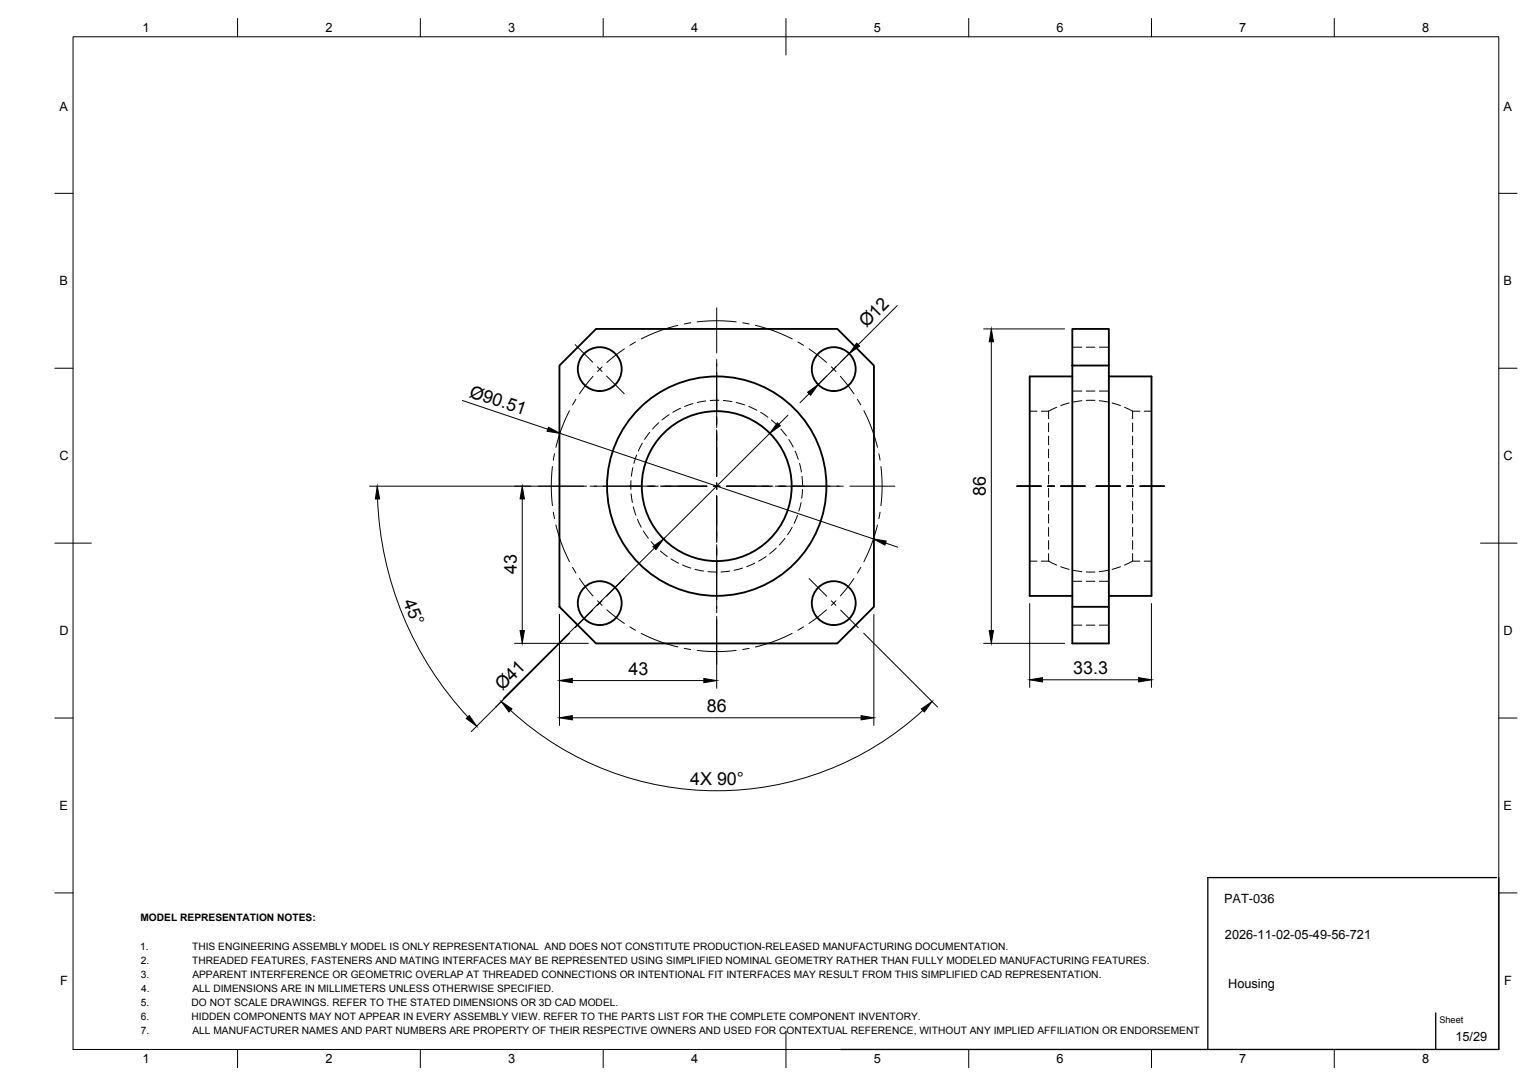
ISO-10303-21;
HEADER;
/* Generated by software containing ST-Developer
 * from STEP Tools, Inc. (www.steptools.com) 
 */

FILE_DESCRIPTION(
/* description */ ('Flange-mounted spindle'),
/* implementation_level */ '2;1');

FILE_NAME(
/* name */ 'Housing.step',
/* time_stamp */ '2026-10-27T10:49:51-07:00',
/* author */ (''),
/* organization */ (''),
/* preprocessor_version */ 'ST-DEVELOPER v20.2',
/* originating_system */ 'Autodesk Translation Framework v15.17.0.0',
/* authorisation */ '');

FILE_SCHEMA (('AUTOMOTIVE_DESIGN { 1 0 10303 214 3 1 1 }'));
ENDSEC;

DATA;
#10=MECHANICAL_DESIGN_GEOMETRIC_PRESENTATION_REPRESENTATION('',(#347),#11764);
#261=SPHERICAL_SURFACE('',#6586,2.35);
#293=SHAPE_REPRESENTATION_RELATIONSHIP('SRR','None',#11890,#320);
#320=ADVANCED_BREP_SHAPE_REPRESENTATION('',(#374),#11745);
#347=STYLED_ITEM('',(#12078),#374);
#374=MANIFOLD_SOLID_BREP('Body1',#6140);
#418=FACE_BOUND('',#1116,.T.);
#419=FACE_BOUND('',#1117,.T.);
#420=FACE_BOUND('',#1121,.T.);
#421=FACE_BOUND('',#1123,.T.);
#422=FACE_BOUND('',#1137,.T.);
#423=FACE_BOUND('',#1138,.T.);
#424=FACE_BOUND('',#1139,.T.);
#425=FACE_BOUND('',#1140,.T.);
#426=FACE_BOUND('',#1141,.T.);
#427=FACE_BOUND('',#1143,.T.);
#428=FACE_BOUND('',#1144,.T.);
#429=FACE_BOUND('',#1145,.T.);
#430=FACE_BOUND('',#1146,.T.);
#431=FACE_BOUND('',#1147,.T.);
#551=PLANE('',#6594);
#552=PLANE('',#6595);
#553=PLANE('',#6608);
#554=PLANE('',#6609);
#555=PLANE('',#6610);
#556=PLANE('',#6611);
#557=PLANE('',#6612);
#558=PLANE('',#6613);
#559=PLANE('',#6614);
#560=PLANE('',#6615);
#561=PLANE('',#6616);
#562=PLANE('',#6617);
#741=FACE_OUTER_BOUND('',#1113,.T.);
#742=FACE_OUTER_BOUND('',#1114,.T.);
#743=FACE_OUTER_BOUND('',#1115,.T.);
#744=FACE_OUTER_BOUND('',#1118,.T.);
#745=FACE_OUTER_BOUND('',#1119,.T.);
#746=FACE_OUTER_BOUND('',#1120,.T.);
#747=FACE_OUTER_BOUND('',#1122,.T.);
#748=FACE_OUTER_BOUND('',#1124,.T.);
#749=FACE_OUTER_BOUND('',#1125,.T.);
#750=FACE_OUTER_BOUND('',#1126,.T.);
#751=FACE_OUTER_BOUND('',#1127,.T.);
#752=FACE_OUTER_BOUND('',#1128,.T.);
#753=FACE_OUTER_BOUND('',#1129,.T.);
#754=FACE_OUTER_BOUND('',#1130,.T.);
#755=FACE_OUTER_BOUND('',#1131,.T.);
#756=FACE_OUTER_BOUND('',#1132,.T.);
#757=FACE_OUTER_BOUND('',#1133,.T.);
#758=FACE_OUTER_BOUND('',#1134,.T.);
#759=FACE_OUTER_BOUND('',#1135,.T.);
#760=FACE_OUTER_BOUND('',#1136,.T.);
#761=FACE_OUTER_BOUND('',#1142,.T.);
#1113=EDGE_LOOP('',(#4275,#4276,#4277,#4278));
#1114=EDGE_LOOP('',(#4279,#4280,#4281,#4282));
#1115=EDGE_LOOP('',(#4283,#4284));
#1116=EDGE_LOOP('',(#4285));
#1117=EDGE_LOOP('',(#4286));
#1118=EDGE_LOOP('',(#4287,#4288,#4289,#4290));
#1119=EDGE_LOOP('',(#4291,#4292,#4293,#4294));
#1120=EDGE_LOOP('',(#4295));
#1121=EDGE_LOOP('',(#4296));
#1122=EDGE_LOOP('',(#4297));
#1123=EDGE_LOOP('',(#4298));
#1124=EDGE_LOOP('',(#4299,#4300,#4301,#4302));
#1125=EDGE_LOOP('',(#4303,#4304,#4305,#4306));
#1126=EDGE_LOOP('',(#4307,#4308,#4309,#4310));
#1127=EDGE_LOOP('',(#4311,#4312,#4313,#4314));
#1128=EDGE_LOOP('',(#4315,#4316,#4317,#4318));
#1129=EDGE_LOOP('',(#4319,#4320,#4321,#4322));
#1130=EDGE_LOOP('',(#4323,#4324,#4325,#4326));
#1131=EDGE_LOOP('',(#4327,#4328,#4329,#4330));
#1132=EDGE_LOOP('',(#4331,#4332,#4333,#4334));
#1133=EDGE_LOOP('',(#4335,#4336,#4337,#4338));
#1134=EDGE_LOOP('',(#4339,#4340,#4341,#4342));
#1135=EDGE_LOOP('',(#4343,#4344,#4345,#4346));
#1136=EDGE_LOOP('',(#4347,#4348,#4349,#4350,#4351,#4352,#4353,#4354));
#1137=EDGE_LOOP('',(#4355));
#1138=EDGE_LOOP('',(#4356));
#1139=EDGE_LOOP('',(#4357));
#1140=EDGE_LOOP('',(#4358));
#1141=EDGE_LOOP('',(#4359));
#1142=EDGE_LOOP('',(#4360,#4361,#4362,#4363,#4364,#4365,#4366,#4367));
#1143=EDGE_LOOP('',(#4368));
#1144=EDGE_LOOP('',(#4369));
#1145=EDGE_LOOP('',(#4370));
#1146=EDGE_LOOP('',(#4371));
#1147=EDGE_LOOP('',(#4372));
#1573=LINE('',#9436,#1995);
#1574=LINE('',#9442,#1996);
#1575=LINE('',#9452,#1997);
#1576=LINE('',#9458,#1998);
#1577=LINE('',#9466,#1999);
#1578=LINE('',#9472,#2000);
#1579=LINE('',#9478,#2001);
#1580=LINE('',#9484,#2002);
#1581=LINE('',#9489,#2003);
#1582=LINE('',#9491,#2004);
#1583=LINE('',#9493,#2005);
#1584=LINE('',#9494,#2006);
#1585=LINE('',#9497,#2007);
#1586=LINE('',#9499,#2008);
#1587=LINE('',#9500,#2009);
#1588=LINE('',#9503,#2010);
#1589=LINE('',#9505,#2011);
#1590=LINE('',#9506,#2012);
#1591=LINE('',#9509,#2013);
#1592=LINE('',#9511,#2014);
#1593=LINE('',#9512,#2015);
#1594=LINE('',#9515,#2016);
#1595=LINE('',#9517,#2017);
#1596=LINE('',#9518,#2018);
#1597=LINE('',#9521,#2019);
#1598=LINE('',#9523,#2020);
#1599=LINE('',#9524,#2021);
#1600=LINE('',#9527,#2022);
#1601=LINE('',#9529,#2023);
#1602=LINE('',#9530,#2024);
#1603=LINE('',#9532,#2025);
#1604=LINE('',#9533,#2026);
#1995=VECTOR('',#7548,2.05);
#1996=VECTOR('',#7555,2.05);
#1997=VECTOR('',#7566,3.);
#1998=VECTOR('',#7573,3.);
#1999=VECTOR('',#7584,0.6);
#2000=VECTOR('',#7591,0.6);
#2001=VECTOR('',#7598,0.6);
#2002=VECTOR('',#7605,0.6);
#2003=VECTOR('',#7610,1.);
#2004=VECTOR('',#7611,1.);
#2005=VECTOR('',#7612,1.);
#2006=VECTOR('',#7613,1.);
#2007=VECTOR('',#7616,1.);
#2008=VECTOR('',#7617,1.);
#2009=VECTOR('',#7618,1.);
#2010=VECTOR('',#7621,1.);
#2011=VECTOR('',#7622,1.);
#2012=VECTOR('',#7623,1.);
#2013=VECTOR('',#7626,1.);
#2014=VECTOR('',#7627,1.);
#2015=VECTOR('',#7628,1.);
#2016=VECTOR('',#7631,1.);
#2017=VECTOR('',#7632,1.);
#2018=VECTOR('',#7633,1.);
#2019=VECTOR('',#7636,1.);
#2020=VECTOR('',#7637,1.);
#2021=VECTOR('',#7638,1.);
#2022=VECTOR('',#7641,1.);
#2023=VECTOR('',#7642,1.);
#2024=VECTOR('',#7643,1.);
#2025=VECTOR('',#7646,1.);
#2026=VECTOR('',#7647,1.);
#2364=CIRCLE('',#6581,2.05);
#2365=CIRCLE('',#6582,2.05);
#2366=CIRCLE('',#6584,2.05);
#2367=CIRCLE('',#6585,2.05);
#2368=CIRCLE('',#6587,2.35);
#2369=CIRCLE('',#6589,3.);
#2370=CIRCLE('',#6590,3.);
#2371=CIRCLE('',#6592,3.);
#2372=CIRCLE('',#6593,3.);
#2373=CIRCLE('',#6597,0.6);
#2374=CIRCLE('',#6598,0.6);
#2375=CIRCLE('',#6600,0.6);
#2376=CIRCLE('',#6601,0.6);
#2377=CIRCLE('',#6603,0.6);
#2378=CIRCLE('',#6604,0.6);
#2379=CIRCLE('',#6606,0.6);
#2380=CIRCLE('',#6607,0.6);
#2738=VERTEX_POINT('',#9433);
#2739=VERTEX_POINT('',#9435);
#2740=VERTEX_POINT('',#9439);
#2741=VERTEX_POINT('',#9441);
#2742=VERTEX_POINT('',#9445);
#2743=VERTEX_POINT('',#9446);
#2744=VERTEX_POINT('',#9449);
#2745=VERTEX_POINT('',#9451);
#2746=VERTEX_POINT('',#9455);
#2747=VERTEX_POINT('',#9457);
#2748=VERTEX_POINT('',#9463);
#2749=VERTEX_POINT('',#9465);
#2750=VERTEX_POINT('',#9469);
#2751=VERTEX_POINT('',#9471);
#2752=VERTEX_POINT('',#9475);
#2753=VERTEX_POINT('',#9477);
#2754=VERTEX_POINT('',#9481);
#2755=VERTEX_POINT('',#9483);
#2756=VERTEX_POINT('',#9487);
#2757=VERTEX_POINT('',#9488);
#2758=VERTEX_POINT('',#9490);
#2759=VERTEX_POINT('',#9492);
#2760=VERTEX_POINT('',#9496);
#2761=VERTEX_POINT('',#9498);
#2762=VERTEX_POINT('',#9502);
#2763=VERTEX_POINT('',#9504);
#2764=VERTEX_POINT('',#9508);
#2765=VERTEX_POINT('',#9510);
#2766=VERTEX_POINT('',#9514);
#2767=VERTEX_POINT('',#9516);
#2768=VERTEX_POINT('',#9520);
#2769=VERTEX_POINT('',#9522);
#2770=VERTEX_POINT('',#9526);
#2771=VERTEX_POINT('',#9528);
#3330=EDGE_CURVE('',#2738,#2738,#2364,.T.);
#3331=EDGE_CURVE('',#2738,#2739,#1573,.T.);
#3332=EDGE_CURVE('',#2739,#2739,#2365,.T.);
#3333=EDGE_CURVE('',#2740,#2740,#2366,.T.);
#3334=EDGE_CURVE('',#2740,#2741,#1574,.T.);
#3335=EDGE_CURVE('',#2741,#2741,#2367,.T.);
#3336=EDGE_CURVE('',#2742,#2743,#2368,.T.);
#3337=EDGE_CURVE('',#2744,#2744,#2369,.T.);
#3338=EDGE_CURVE('',#2744,#2745,#1575,.T.);
#3339=EDGE_CURVE('',#2745,#2745,#2370,.T.);
#3340=EDGE_CURVE('',#2746,#2746,#2371,.T.);
#3341=EDGE_CURVE('',#2746,#2747,#1576,.T.);
#3342=EDGE_CURVE('',#2747,#2747,#2372,.T.);
#3343=EDGE_CURVE('',#2748,#2748,#2373,.T.);
#3344=EDGE_CURVE('',#2748,#2749,#1577,.T.);
#3345=EDGE_CURVE('',#2749,#2749,#2374,.T.);
#3346=EDGE_CURVE('',#2750,#2750,#2375,.T.);
#3347=EDGE_CURVE('',#2750,#2751,#1578,.T.);
#3348=EDGE_CURVE('',#2751,#2751,#2376,.T.);
#3349=EDGE_CURVE('',#2752,#2752,#2377,.T.);
#3350=EDGE_CURVE('',#2752,#2753,#1579,.T.);
#3351=EDGE_CURVE('',#2753,#2753,#2378,.T.);
#3352=EDGE_CURVE('',#2754,#2754,#2379,.T.);
#3353=EDGE_CURVE('',#2754,#2755,#1580,.T.);
#3354=EDGE_CURVE('',#2755,#2755,#2380,.T.);
#3355=EDGE_CURVE('',#2756,#2757,#1581,.T.);
#3356=EDGE_CURVE('',#2757,#2758,#1582,.T.);
#3357=EDGE_CURVE('',#2759,#2758,#1583,.T.);
#3358=EDGE_CURVE('',#2756,#2759,#1584,.T.);
#3359=EDGE_CURVE('',#2760,#2756,#1585,.T.);
#3360=EDGE_CURVE('',#2761,#2759,#1586,.T.);
#3361=EDGE_CURVE('',#2760,#2761,#1587,.T.);
#3362=EDGE_CURVE('',#2762,#2760,#1588,.T.);
#3363=EDGE_CURVE('',#2763,#2761,#1589,.T.);
#3364=EDGE_CURVE('',#2762,#2763,#1590,.T.);
#3365=EDGE_CURVE('',#2764,#2762,#1591,.T.);
#3366=EDGE_CURVE('',#2765,#2763,#1592,.T.);
#3367=EDGE_CURVE('',#2764,#2765,#1593,.T.);
#3368=EDGE_CURVE('',#2766,#2764,#1594,.T.);
#3369=EDGE_CURVE('',#2767,#2765,#1595,.T.);
#3370=EDGE_CURVE('',#2766,#2767,#1596,.T.);
#3371=EDGE_CURVE('',#2768,#2766,#1597,.T.);
#3372=EDGE_CURVE('',#2769,#2767,#1598,.T.);
#3373=EDGE_CURVE('',#2768,#2769,#1599,.T.);
#3374=EDGE_CURVE('',#2770,#2768,#1600,.T.);
#3375=EDGE_CURVE('',#2771,#2769,#1601,.T.);
#3376=EDGE_CURVE('',#2770,#2771,#1602,.T.);
#3377=EDGE_CURVE('',#2757,#2770,#1603,.T.);
#3378=EDGE_CURVE('',#2758,#2771,#1604,.T.);
#4275=ORIENTED_EDGE('',*,*,#3330,.F.);
#4276=ORIENTED_EDGE('',*,*,#3331,.T.);
#4277=ORIENTED_EDGE('',*,*,#3332,.F.);
#4278=ORIENTED_EDGE('',*,*,#3331,.F.);
#4279=ORIENTED_EDGE('',*,*,#3333,.F.);
#4280=ORIENTED_EDGE('',*,*,#3334,.T.);
#4281=ORIENTED_EDGE('',*,*,#3335,.F.);
#4282=ORIENTED_EDGE('',*,*,#3334,.F.);
#4283=ORIENTED_EDGE('',*,*,#3336,.T.);
#4284=ORIENTED_EDGE('',*,*,#3336,.F.);
#4285=ORIENTED_EDGE('',*,*,#3333,.T.);
#4286=ORIENTED_EDGE('',*,*,#3332,.T.);
#4287=ORIENTED_EDGE('',*,*,#3337,.F.);
#4288=ORIENTED_EDGE('',*,*,#3338,.T.);
#4289=ORIENTED_EDGE('',*,*,#3339,.F.);
#4290=ORIENTED_EDGE('',*,*,#3338,.F.);
#4291=ORIENTED_EDGE('',*,*,#3340,.F.);
#4292=ORIENTED_EDGE('',*,*,#3341,.T.);
#4293=ORIENTED_EDGE('',*,*,#3342,.F.);
#4294=ORIENTED_EDGE('',*,*,#3341,.F.);
#4295=ORIENTED_EDGE('',*,*,#3339,.T.);
#4296=ORIENTED_EDGE('',*,*,#3330,.T.);
#4297=ORIENTED_EDGE('',*,*,#3340,.T.);
#4298=ORIENTED_EDGE('',*,*,#3335,.T.);
#4299=ORIENTED_EDGE('',*,*,#3343,.F.);
#4300=ORIENTED_EDGE('',*,*,#3344,.T.);
#4301=ORIENTED_EDGE('',*,*,#3345,.F.);
#4302=ORIENTED_EDGE('',*,*,#3344,.F.);
#4303=ORIENTED_EDGE('',*,*,#3346,.F.);
#4304=ORIENTED_EDGE('',*,*,#3347,.T.);
#4305=ORIENTED_EDGE('',*,*,#3348,.F.);
#4306=ORIENTED_EDGE('',*,*,#3347,.F.);
#4307=ORIENTED_EDGE('',*,*,#3349,.F.);
#4308=ORIENTED_EDGE('',*,*,#3350,.T.);
#4309=ORIENTED_EDGE('',*,*,#3351,.F.);
#4310=ORIENTED_EDGE('',*,*,#3350,.F.);
#4311=ORIENTED_EDGE('',*,*,#3352,.F.);
#4312=ORIENTED_EDGE('',*,*,#3353,.T.);
#4313=ORIENTED_EDGE('',*,*,#3354,.F.);
#4314=ORIENTED_EDGE('',*,*,#3353,.F.);
#4315=ORIENTED_EDGE('',*,*,#3355,.T.);
#4316=ORIENTED_EDGE('',*,*,#3356,.T.);
#4317=ORIENTED_EDGE('',*,*,#3357,.F.);
#4318=ORIENTED_EDGE('',*,*,#3358,.F.);
#4319=ORIENTED_EDGE('',*,*,#3359,.T.);
#4320=ORIENTED_EDGE('',*,*,#3358,.T.);
#4321=ORIENTED_EDGE('',*,*,#3360,.F.);
#4322=ORIENTED_EDGE('',*,*,#3361,.F.);
#4323=ORIENTED_EDGE('',*,*,#3362,.T.);
#4324=ORIENTED_EDGE('',*,*,#3361,.T.);
#4325=ORIENTED_EDGE('',*,*,#3363,.F.);
#4326=ORIENTED_EDGE('',*,*,#3364,.F.);
#4327=ORIENTED_EDGE('',*,*,#3365,.T.);
#4328=ORIENTED_EDGE('',*,*,#3364,.T.);
#4329=ORIENTED_EDGE('',*,*,#3366,.F.);
#4330=ORIENTED_EDGE('',*,*,#3367,.F.);
#4331=ORIENTED_EDGE('',*,*,#3368,.T.);
#4332=ORIENTED_EDGE('',*,*,#3367,.T.);
#4333=ORIENTED_EDGE('',*,*,#3369,.F.);
#4334=ORIENTED_EDGE('',*,*,#3370,.F.);
#4335=ORIENTED_EDGE('',*,*,#3371,.T.);
#4336=ORIENTED_EDGE('',*,*,#3370,.T.);
#4337=ORIENTED_EDGE('',*,*,#3372,.F.);
#4338=ORIENTED_EDGE('',*,*,#3373,.F.);
#4339=ORIENTED_EDGE('',*,*,#3374,.T.);
#4340=ORIENTED_EDGE('',*,*,#3373,.T.);
#4341=ORIENTED_EDGE('',*,*,#3375,.F.);
#4342=ORIENTED_EDGE('',*,*,#3376,.F.);
#4343=ORIENTED_EDGE('',*,*,#3377,.T.);
#4344=ORIENTED_EDGE('',*,*,#3376,.T.);
#4345=ORIENTED_EDGE('',*,*,#3378,.F.);
#4346=ORIENTED_EDGE('',*,*,#3356,.F.);
#4347=ORIENTED_EDGE('',*,*,#3378,.T.);
#4348=ORIENTED_EDGE('',*,*,#3375,.T.);
#4349=ORIENTED_EDGE('',*,*,#3372,.T.);
#4350=ORIENTED_EDGE('',*,*,#3369,.T.);
#4351=ORIENTED_EDGE('',*,*,#3366,.T.);
#4352=ORIENTED_EDGE('',*,*,#3363,.T.);
#4353=ORIENTED_EDGE('',*,*,#3360,.T.);
#4354=ORIENTED_EDGE('',*,*,#3357,.T.);
#4355=ORIENTED_EDGE('',*,*,#3342,.T.);
#4356=ORIENTED_EDGE('',*,*,#3345,.T.);
#4357=ORIENTED_EDGE('',*,*,#3348,.T.);
#4358=ORIENTED_EDGE('',*,*,#3351,.T.);
#4359=ORIENTED_EDGE('',*,*,#3354,.T.);
#4360=ORIENTED_EDGE('',*,*,#3377,.F.);
#4361=ORIENTED_EDGE('',*,*,#3355,.F.);
#4362=ORIENTED_EDGE('',*,*,#3359,.F.);
#4363=ORIENTED_EDGE('',*,*,#3362,.F.);
#4364=ORIENTED_EDGE('',*,*,#3365,.F.);
#4365=ORIENTED_EDGE('',*,*,#3368,.F.);
#4366=ORIENTED_EDGE('',*,*,#3371,.F.);
#4367=ORIENTED_EDGE('',*,*,#3374,.F.);
#4368=ORIENTED_EDGE('',*,*,#3337,.T.);
#4369=ORIENTED_EDGE('',*,*,#3343,.T.);
#4370=ORIENTED_EDGE('',*,*,#3346,.T.);
#4371=ORIENTED_EDGE('',*,*,#3349,.T.);
#4372=ORIENTED_EDGE('',*,*,#3352,.T.);
#5644=CYLINDRICAL_SURFACE('',#6580,2.05);
#5645=CYLINDRICAL_SURFACE('',#6583,2.05);
#5646=CYLINDRICAL_SURFACE('',#6588,3.);
#5647=CYLINDRICAL_SURFACE('',#6591,3.);
#5648=CYLINDRICAL_SURFACE('',#6596,0.6);
#5649=CYLINDRICAL_SURFACE('',#6599,0.6);
#5650=CYLINDRICAL_SURFACE('',#6602,0.6);
#5651=CYLINDRICAL_SURFACE('',#6605,0.6);
#5852=ADVANCED_FACE('',(#741),#5644,.F.);
#5853=ADVANCED_FACE('',(#742),#5645,.F.);
#5854=ADVANCED_FACE('',(#743,#418,#419),#261,.F.);
#5855=ADVANCED_FACE('',(#744),#5646,.T.);
#5856=ADVANCED_FACE('',(#745),#5647,.T.);
#5857=ADVANCED_FACE('',(#746,#420),#551,.F.);
#5858=ADVANCED_FACE('',(#747,#421),#552,.T.);
#5859=ADVANCED_FACE('',(#748),#5648,.F.);
#5860=ADVANCED_FACE('',(#749),#5649,.F.);
#5861=ADVANCED_FACE('',(#750),#5650,.F.);
#5862=ADVANCED_FACE('',(#751),#5651,.F.);
#5863=ADVANCED_FACE('',(#752),#553,.T.);
#5864=ADVANCED_FACE('',(#753),#554,.T.);
#5865=ADVANCED_FACE('',(#754),#555,.T.);
#5866=ADVANCED_FACE('',(#755),#556,.T.);
#5867=ADVANCED_FACE('',(#756),#557,.T.);
#5868=ADVANCED_FACE('',(#757),#558,.T.);
#5869=ADVANCED_FACE('',(#758),#559,.T.);
#5870=ADVANCED_FACE('',(#759),#560,.T.);
#5871=ADVANCED_FACE('',(#760,#422,#423,#424,#425,#426),#561,.T.);
#5872=ADVANCED_FACE('',(#761,#427,#428,#429,#430,#431),#562,.F.);
#6140=CLOSED_SHELL('',(#5852,#5853,#5854,#5855,#5856,#5857,#5858,#5859,
#5860,#5861,#5862,#5863,#5864,#5865,#5866,#5867,#5868,#5869,#5870,#5871,
#5872));
#6579=AXIS2_PLACEMENT_3D('',#9431,#7542,#7543);
#6580=AXIS2_PLACEMENT_3D('',#9432,#7544,#7545);
#6581=AXIS2_PLACEMENT_3D('',#9434,#7546,#7547);
#6582=AXIS2_PLACEMENT_3D('',#9437,#7549,#7550);
#6583=AXIS2_PLACEMENT_3D('',#9438,#7551,#7552);
#6584=AXIS2_PLACEMENT_3D('',#9440,#7553,#7554);
#6585=AXIS2_PLACEMENT_3D('',#9443,#7556,#7557);
#6586=AXIS2_PLACEMENT_3D('',#9444,#7558,#7559);
#6587=AXIS2_PLACEMENT_3D('',#9447,#7560,#7561);
#6588=AXIS2_PLACEMENT_3D('',#9448,#7562,#7563);
#6589=AXIS2_PLACEMENT_3D('',#9450,#7564,#7565);
#6590=AXIS2_PLACEMENT_3D('',#9453,#7567,#7568);
#6591=AXIS2_PLACEMENT_3D('',#9454,#7569,#7570);
#6592=AXIS2_PLACEMENT_3D('',#9456,#7571,#7572);
#6593=AXIS2_PLACEMENT_3D('',#9459,#7574,#7575);
#6594=AXIS2_PLACEMENT_3D('',#9460,#7576,#7577);
#6595=AXIS2_PLACEMENT_3D('',#9461,#7578,#7579);
#6596=AXIS2_PLACEMENT_3D('',#9462,#7580,#7581);
#6597=AXIS2_PLACEMENT_3D('',#9464,#7582,#7583);
#6598=AXIS2_PLACEMENT_3D('',#9467,#7585,#7586);
#6599=AXIS2_PLACEMENT_3D('',#9468,#7587,#7588);
#6600=AXIS2_PLACEMENT_3D('',#9470,#7589,#7590);
#6601=AXIS2_PLACEMENT_3D('',#9473,#7592,#7593);
#6602=AXIS2_PLACEMENT_3D('',#9474,#7594,#7595);
#6603=AXIS2_PLACEMENT_3D('',#9476,#7596,#7597);
#6604=AXIS2_PLACEMENT_3D('',#9479,#7599,#7600);
#6605=AXIS2_PLACEMENT_3D('',#9480,#7601,#7602);
#6606=AXIS2_PLACEMENT_3D('',#9482,#7603,#7604);
#6607=AXIS2_PLACEMENT_3D('',#9485,#7606,#7607);
#6608=AXIS2_PLACEMENT_3D('',#9486,#7608,#7609);
#6609=AXIS2_PLACEMENT_3D('',#9495,#7614,#7615);
#6610=AXIS2_PLACEMENT_3D('',#9501,#7619,#7620);
#6611=AXIS2_PLACEMENT_3D('',#9507,#7624,#7625);
#6612=AXIS2_PLACEMENT_3D('',#9513,#7629,#7630);
#6613=AXIS2_PLACEMENT_3D('',#9519,#7634,#7635);
#6614=AXIS2_PLACEMENT_3D('',#9525,#7639,#7640);
#6615=AXIS2_PLACEMENT_3D('',#9531,#7644,#7645);
#6616=AXIS2_PLACEMENT_3D('',#9534,#7648,#7649);
#6617=AXIS2_PLACEMENT_3D('',#9535,#7650,#7651);
#7542=DIRECTION('axis',(0.,0.,1.));
#7543=DIRECTION('refdir',(1.,0.,0.));
#7544=DIRECTION('center_axis',(0.,1.,0.));
#7545=DIRECTION('ref_axis',(1.,0.,0.));
#7546=DIRECTION('center_axis',(0.,1.,0.));
#7547=DIRECTION('ref_axis',(1.,0.,0.));
#7548=DIRECTION('',(0.,1.,0.));
#7549=DIRECTION('center_axis',(0.,-1.,0.));
#7550=DIRECTION('ref_axis',(1.,0.,0.));
#7551=DIRECTION('center_axis',(0.,1.,0.));
#7552=DIRECTION('ref_axis',(1.,0.,0.));
#7553=DIRECTION('center_axis',(0.,1.,0.));
#7554=DIRECTION('ref_axis',(1.,0.,0.));
#7555=DIRECTION('',(0.,1.,0.));
#7556=DIRECTION('center_axis',(0.,-1.,0.));
#7557=DIRECTION('ref_axis',(1.,0.,0.));
#7558=DIRECTION('center_axis',(6.12323399573677E-17,0.,1.));
#7559=DIRECTION('ref_axis',(1.,0.,0.));
#7560=DIRECTION('center_axis',(-1.22464679914735E-16,1.,0.));
#7561=DIRECTION('ref_axis',(-1.,-1.22464679914735E-16,0.));
#7562=DIRECTION('center_axis',(0.,1.,0.));
#7563=DIRECTION('ref_axis',(1.,0.,0.));
#7564=DIRECTION('center_axis',(0.,1.,0.));
#7565=DIRECTION('ref_axis',(1.,0.,0.));
#7566=DIRECTION('',(0.,-1.,0.));
#7567=DIRECTION('center_axis',(0.,-1.,0.));
#7568=DIRECTION('ref_axis',(1.,0.,0.));
#7569=DIRECTION('center_axis',(0.,1.,0.));
#7570=DIRECTION('ref_axis',(1.,0.,0.));
#7571=DIRECTION('center_axis',(0.,1.,0.));
#7572=DIRECTION('ref_axis',(1.,0.,0.));
#7573=DIRECTION('',(0.,-1.,0.));
#7574=DIRECTION('center_axis',(0.,-1.,0.));
#7575=DIRECTION('ref_axis',(1.,0.,0.));
#7576=DIRECTION('center_axis',(0.,1.,0.));
#7577=DIRECTION('ref_axis',(1.,0.,0.));
#7578=DIRECTION('center_axis',(0.,1.,0.));
#7579=DIRECTION('ref_axis',(1.,0.,0.));
#7580=DIRECTION('center_axis',(0.,1.,0.));
#7581=DIRECTION('ref_axis',(1.,0.,0.));
#7582=DIRECTION('center_axis',(0.,1.,0.));
#7583=DIRECTION('ref_axis',(1.,0.,0.));
#7584=DIRECTION('',(0.,1.,0.));
#7585=DIRECTION('center_axis',(0.,-1.,0.));
#7586=DIRECTION('ref_axis',(1.,0.,0.));
#7587=DIRECTION('center_axis',(0.,1.,0.));
#7588=DIRECTION('ref_axis',(1.,0.,0.));
#7589=DIRECTION('center_axis',(0.,1.,0.));
#7590=DIRECTION('ref_axis',(1.,0.,0.));
#7591=DIRECTION('',(0.,1.,0.));
#7592=DIRECTION('center_axis',(0.,-1.,0.));
#7593=DIRECTION('ref_axis',(1.,0.,0.));
#7594=DIRECTION('center_axis',(0.,1.,0.));
#7595=DIRECTION('ref_axis',(1.,0.,0.));
#7596=DIRECTION('center_axis',(0.,1.,0.));
#7597=DIRECTION('ref_axis',(1.,0.,0.));
#7598=DIRECTION('',(0.,1.,0.));
#7599=DIRECTION('center_axis',(0.,-1.,0.));
#7600=DIRECTION('ref_axis',(1.,0.,0.));
#7601=DIRECTION('center_axis',(0.,1.,0.));
#7602=DIRECTION('ref_axis',(1.,0.,0.));
#7603=DIRECTION('center_axis',(0.,1.,0.));
#7604=DIRECTION('ref_axis',(1.,0.,0.));
#7605=DIRECTION('',(0.,1.,0.));
#7606=DIRECTION('center_axis',(0.,-1.,0.));
#7607=DIRECTION('ref_axis',(1.,0.,0.));
#7608=DIRECTION('center_axis',(-1.,0.,0.));
#7609=DIRECTION('ref_axis',(0.,0.,1.));
#7610=DIRECTION('',(0.,0.,1.));
#7611=DIRECTION('',(0.,1.,0.));
#7612=DIRECTION('',(0.,0.,1.));
#7613=DIRECTION('',(0.,1.,0.));
#7614=DIRECTION('center_axis',(-0.707106781186548,0.,-0.707106781186548));
#7615=DIRECTION('ref_axis',(-0.707106781186548,0.,0.707106781186548));
#7616=DIRECTION('',(-0.707106781186548,0.,0.707106781186548));
#7617=DIRECTION('',(-0.707106781186548,0.,0.707106781186548));
#7618=DIRECTION('',(0.,1.,0.));
#7619=DIRECTION('center_axis',(0.,0.,-1.));
#7620=DIRECTION('ref_axis',(-1.,0.,0.));
#7621=DIRECTION('',(-1.,0.,0.));
#7622=DIRECTION('',(-1.,0.,0.));
#7623=DIRECTION('',(0.,1.,0.));
#7624=DIRECTION('center_axis',(0.707106781186548,0.,-0.707106781186548));
#7625=DIRECTION('ref_axis',(-0.707106781186548,0.,-0.707106781186548));
#7626=DIRECTION('',(-0.707106781186548,0.,-0.707106781186548));
#7627=DIRECTION('',(-0.707106781186548,0.,-0.707106781186548));
#7628=DIRECTION('',(0.,1.,0.));
#7629=DIRECTION('center_axis',(1.,0.,0.));
#7630=DIRECTION('ref_axis',(0.,0.,-1.));
#7631=DIRECTION('',(0.,0.,-1.));
#7632=DIRECTION('',(0.,0.,-1.));
#7633=DIRECTION('',(0.,1.,0.));
#7634=DIRECTION('center_axis',(0.707106781186548,0.,0.707106781186548));
#7635=DIRECTION('ref_axis',(0.707106781186548,0.,-0.707106781186548));
#7636=DIRECTION('',(0.707106781186548,0.,-0.707106781186548));
#7637=DIRECTION('',(0.707106781186548,0.,-0.707106781186548));
#7638=DIRECTION('',(0.,1.,0.));
#7639=DIRECTION('center_axis',(0.,0.,1.));
#7640=DIRECTION('ref_axis',(1.,0.,0.));
#7641=DIRECTION('',(1.,0.,0.));
#7642=DIRECTION('',(1.,0.,0.));
#7643=DIRECTION('',(0.,1.,0.));
#7644=DIRECTION('center_axis',(-0.707106781186548,0.,0.707106781186548));
#7645=DIRECTION('ref_axis',(0.707106781186548,0.,0.707106781186548));
#7646=DIRECTION('',(0.707106781186548,0.,0.707106781186548));
#7647=DIRECTION('',(0.707106781186548,0.,0.707106781186548));
#7648=DIRECTION('center_axis',(0.,1.,0.));
#7649=DIRECTION('ref_axis',(0.,0.,1.));
#7650=DIRECTION('center_axis',(0.,1.,0.));
#7651=DIRECTION('ref_axis',(1.,0.,0.));
#9431=CARTESIAN_POINT('',(0.,0.,0.));
#9432=CARTESIAN_POINT('Origin',(0.,0.,0.));
#9433=CARTESIAN_POINT('',(-2.05,-1.665,2.51052593825207E-16));
#9434=CARTESIAN_POINT('Origin',(0.,-1.665,0.));
#9435=CARTESIAN_POINT('',(-2.05,-1.14891252930761,-2.51052593825207E-16));
#9436=CARTESIAN_POINT('',(-2.05,0.,2.51052593825207E-16));
#9437=CARTESIAN_POINT('Origin',(0.,-1.14891252930761,0.));
#9438=CARTESIAN_POINT('Origin',(0.,0.,0.));
#9439=CARTESIAN_POINT('',(-2.05,1.14891252930761,2.51052593825207E-16));
#9440=CARTESIAN_POINT('Origin',(0.,1.14891252930761,0.));
#9441=CARTESIAN_POINT('',(-2.05,1.665,-2.51052593825207E-16));
#9442=CARTESIAN_POINT('',(-2.05,0.,2.51052593825207E-16));
#9443=CARTESIAN_POINT('Origin',(0.,1.665,0.));
#9444=CARTESIAN_POINT('Origin',(0.,0.,0.));
#9445=CARTESIAN_POINT('',(-1.43895998899814E-16,-1.76221774462768E-32,-2.35));
#9446=CARTESIAN_POINT('',(-1.43895998899814E-16,-1.76221774462768E-32,2.35));
#9447=CARTESIAN_POINT('Origin',(0.,0.,0.));
#9448=CARTESIAN_POINT('Origin',(0.,0.,0.));
#9449=CARTESIAN_POINT('',(-3.,-0.5,3.67394039744206E-16));
#9450=CARTESIAN_POINT('Origin',(0.,-0.5,0.));
#9451=CARTESIAN_POINT('',(-3.,-1.665,3.67394039744206E-16));
#9452=CARTESIAN_POINT('',(-3.,0.,3.67394039744206E-16));
#9453=CARTESIAN_POINT('Origin',(0.,-1.665,0.));
#9454=CARTESIAN_POINT('Origin',(0.,0.,0.));
#9455=CARTESIAN_POINT('',(-3.,1.665,3.67394039744206E-16));
#9456=CARTESIAN_POINT('Origin',(0.,1.665,0.));
#9457=CARTESIAN_POINT('',(-3.,0.5,-3.67394039744206E-16));
#9458=CARTESIAN_POINT('',(-3.,0.,3.67394039744206E-16));
#9459=CARTESIAN_POINT('Origin',(0.,0.5,0.));
#9460=CARTESIAN_POINT('Origin',(0.,-1.665,0.));
#9461=CARTESIAN_POINT('Origin',(0.,1.665,0.));
#9462=CARTESIAN_POINT('Origin',(3.2,0.,3.2));
#9463=CARTESIAN_POINT('',(2.6,-0.5,3.2));
#9464=CARTESIAN_POINT('Origin',(3.2,-0.5,3.2));
#9465=CARTESIAN_POINT('',(2.6,0.5,3.2));
#9466=CARTESIAN_POINT('',(2.6,0.,3.2));
#9467=CARTESIAN_POINT('Origin',(3.2,0.5,3.2));
#9468=CARTESIAN_POINT('Origin',(-3.2,0.,-3.2));
#9469=CARTESIAN_POINT('',(-3.8,-0.5,-3.2));
#9470=CARTESIAN_POINT('Origin',(-3.2,-0.5,-3.2));
#9471=CARTESIAN_POINT('',(-3.8,0.5,-3.2));
#9472=CARTESIAN_POINT('',(-3.8,0.,-3.2));
#9473=CARTESIAN_POINT('Origin',(-3.2,0.5,-3.2));
#9474=CARTESIAN_POINT('Origin',(-3.2,0.,3.2));
#9475=CARTESIAN_POINT('',(-3.8,-0.5,3.2));
#9476=CARTESIAN_POINT('Origin',(-3.2,-0.5,3.2));
#9477=CARTESIAN_POINT('',(-3.8,0.5,3.2));
#9478=CARTESIAN_POINT('',(-3.8,0.,3.2));
#9479=CARTESIAN_POINT('Origin',(-3.2,0.5,3.2));
#9480=CARTESIAN_POINT('Origin',(3.2,0.,-3.2));
#9481=CARTESIAN_POINT('',(2.6,-0.5,-3.2));
#9482=CARTESIAN_POINT('Origin',(3.2,-0.5,-3.2));
#9483=CARTESIAN_POINT('',(2.6,0.5,-3.2));
#9484=CARTESIAN_POINT('',(2.6,0.,-3.2));
#9485=CARTESIAN_POINT('Origin',(3.2,0.5,-3.2));
#9486=CARTESIAN_POINT('Origin',(-4.3,-0.5,-3.3));
#9487=CARTESIAN_POINT('',(-4.3,-0.5,-3.3));
#9488=CARTESIAN_POINT('',(-4.3,-0.5,3.3));
#9489=CARTESIAN_POINT('',(-4.3,-0.5,-3.3));
#9490=CARTESIAN_POINT('',(-4.3,0.5,3.3));
#9491=CARTESIAN_POINT('',(-4.3,-0.5,3.3));
#9492=CARTESIAN_POINT('',(-4.3,0.5,-3.3));
#9493=CARTESIAN_POINT('',(-4.3,0.5,-3.3));
#9494=CARTESIAN_POINT('',(-4.3,-0.5,-3.3));
#9495=CARTESIAN_POINT('Origin',(-3.3,-0.5,-4.3));
#9496=CARTESIAN_POINT('',(-3.3,-0.5,-4.3));
#9497=CARTESIAN_POINT('',(-3.3,-0.5,-4.3));
#9498=CARTESIAN_POINT('',(-3.3,0.5,-4.3));
#9499=CARTESIAN_POINT('',(-3.3,0.5,-4.3));
#9500=CARTESIAN_POINT('',(-3.3,-0.5,-4.3));
#9501=CARTESIAN_POINT('Origin',(3.3,-0.5,-4.3));
#9502=CARTESIAN_POINT('',(3.3,-0.5,-4.3));
#9503=CARTESIAN_POINT('',(3.3,-0.5,-4.3));
#9504=CARTESIAN_POINT('',(3.3,0.5,-4.3));
#9505=CARTESIAN_POINT('',(3.3,0.5,-4.3));
#9506=CARTESIAN_POINT('',(3.3,-0.5,-4.3));
#9507=CARTESIAN_POINT('Origin',(4.3,-0.5,-3.3));
#9508=CARTESIAN_POINT('',(4.3,-0.5,-3.3));
#9509=CARTESIAN_POINT('',(4.3,-0.5,-3.3));
#9510=CARTESIAN_POINT('',(4.3,0.5,-3.3));
#9511=CARTESIAN_POINT('',(4.3,0.5,-3.3));
#9512=CARTESIAN_POINT('',(4.3,-0.5,-3.3));
#9513=CARTESIAN_POINT('Origin',(4.3,-0.5,3.3));
#9514=CARTESIAN_POINT('',(4.3,-0.5,3.3));
#9515=CARTESIAN_POINT('',(4.3,-0.5,3.3));
#9516=CARTESIAN_POINT('',(4.3,0.5,3.3));
#9517=CARTESIAN_POINT('',(4.3,0.5,3.3));
#9518=CARTESIAN_POINT('',(4.3,-0.5,3.3));
#9519=CARTESIAN_POINT('Origin',(3.3,-0.5,4.3));
#9520=CARTESIAN_POINT('',(3.3,-0.5,4.3));
#9521=CARTESIAN_POINT('',(3.3,-0.5,4.3));
#9522=CARTESIAN_POINT('',(3.3,0.5,4.3));
#9523=CARTESIAN_POINT('',(3.3,0.5,4.3));
#9524=CARTESIAN_POINT('',(3.3,-0.5,4.3));
#9525=CARTESIAN_POINT('Origin',(-3.3,-0.5,4.3));
#9526=CARTESIAN_POINT('',(-3.3,-0.5,4.3));
#9527=CARTESIAN_POINT('',(-3.3,-0.5,4.3));
#9528=CARTESIAN_POINT('',(-3.3,0.5,4.3));
#9529=CARTESIAN_POINT('',(-3.3,0.5,4.3));
#9530=CARTESIAN_POINT('',(-3.3,-0.5,4.3));
#9531=CARTESIAN_POINT('Origin',(-4.3,-0.5,3.3));
#9532=CARTESIAN_POINT('',(-4.3,-0.5,3.3));
#9533=CARTESIAN_POINT('',(-4.3,0.5,3.3));
#9534=CARTESIAN_POINT('Origin',(0.,0.5,0.));
#9535=CARTESIAN_POINT('Origin',(0.,-0.5,0.));
#11713=UNCERTAINTY_MEASURE_WITH_UNIT(LENGTH_MEASURE(0.001),#11765,
'DISTANCE_ACCURACY_VALUE',
'Maximum model space distance between geometric entities at asserted c
onnectivities');
#11732=UNCERTAINTY_MEASURE_WITH_UNIT(LENGTH_MEASURE(0.001),#11765,
'DISTANCE_ACCURACY_VALUE',
'Maximum model space distance between geometric entities at asserted c
onnectivities');
#11745=(
GEOMETRIC_REPRESENTATION_CONTEXT(3)
GLOBAL_UNCERTAINTY_ASSIGNED_CONTEXT((#11713))
GLOBAL_UNIT_ASSIGNED_CONTEXT((#11765,#11767,#11768))
REPRESENTATION_CONTEXT('','3D')
);
#11764=(
GEOMETRIC_REPRESENTATION_CONTEXT(3)
GLOBAL_UNCERTAINTY_ASSIGNED_CONTEXT((#11732))
GLOBAL_UNIT_ASSIGNED_CONTEXT((#11765,#11767,#11768))
REPRESENTATION_CONTEXT('','3D')
);
#11765=(
LENGTH_UNIT()
NAMED_UNIT(*)
SI_UNIT(.CENTI.,.METRE.)
);
#11767=(
NAMED_UNIT(*)
PLANE_ANGLE_UNIT()
SI_UNIT($,.RADIAN.)
);
#11768=(
NAMED_UNIT(*)
SI_UNIT($,.STERADIAN.)
SOLID_ANGLE_UNIT()
);
#11781=SHAPE_DEFINITION_REPRESENTATION(#11812,#11890);
#11812=PRODUCT_DEFINITION_SHAPE('',$,#11922);
#11890=SHAPE_REPRESENTATION('',(#6579),#11745);
#11909=PRODUCT_DEFINITION_CONTEXT('part definition',#12004,'design');
#11922=PRODUCT_DEFINITION('Housing','Housing',#11953,#11909);
#11953=PRODUCT_DEFINITION_FORMATION('',$,#12018);
#12004=APPLICATION_CONTEXT(
'Core Data for Automotive Mechanical Design Process');
#12005=PRODUCT_CONTEXT('part definition',#12004,'mechanical');
#12018=PRODUCT('Housing','Housing','Housing',(#12005));
#12072=COLOUR_RGB('Dark Blue',0.08,0.2,0.34);
#12073=FILL_AREA_STYLE_COLOUR('',#12072);
#12074=FILL_AREA_STYLE('',(#12073));
#12075=SURFACE_STYLE_FILL_AREA(#12074);
#12076=SURFACE_SIDE_STYLE('',(#12075));
#12077=SURFACE_STYLE_USAGE(.BOTH.,#12076);
#12078=PRESENTATION_STYLE_ASSIGNMENT((#12077));
ENDSEC;
END-ISO-10303-21;
